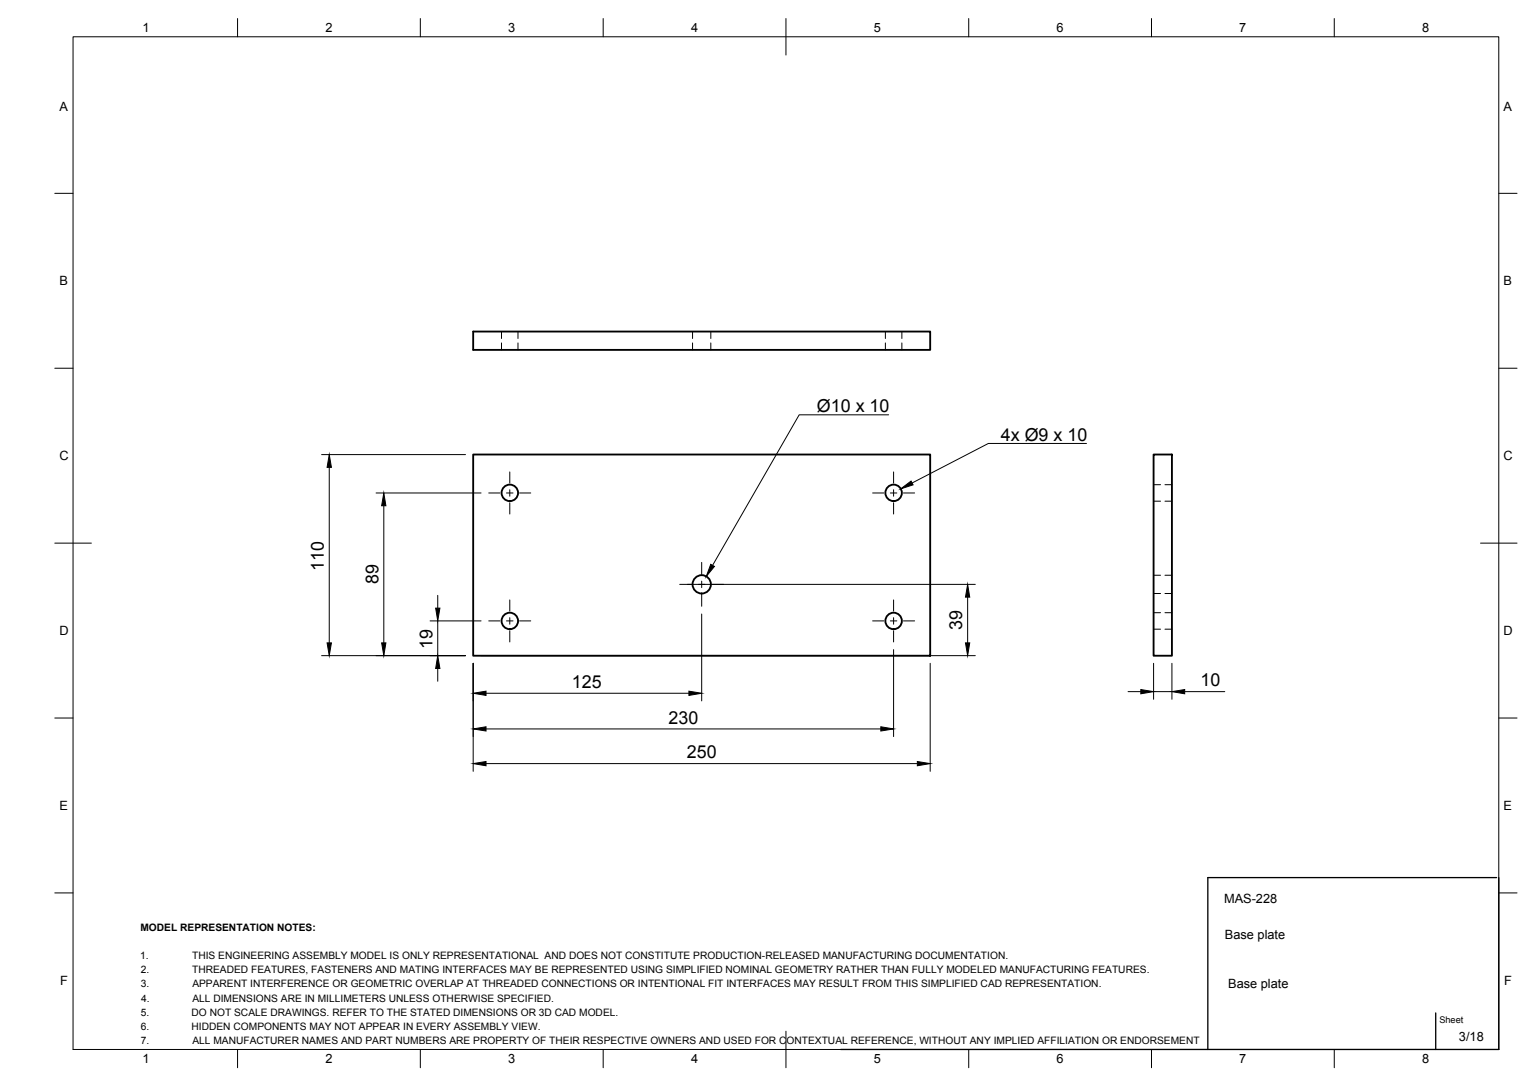
ISO-10303-21;
HEADER;
/* Generated by software containing ST-Developer
 * from STEP Tools, Inc. (www.steptools.com) 
 */

FILE_DESCRIPTION(
/* description */ ('Independent Peaucellier-Lipkin straight-line linkage. Radius arms 100
 mm, inversion-cell links 60 mm, crank radius and fixed-pivot spacing 
32 mm. Inversion constant 6400 mm squared, nominal output straight lin
e X=100 mm. Overhead bearing bridge clears the layered moving links. N
o accuracy or load rating assigned.'),
/* implementation_level */ '2;1');

FILE_NAME(
/* name */ 'Base plate.step',
/* time_stamp */ '2026-11-09T18:06:16-08:00',
/* author */ (''),
/* organization */ (''),
/* preprocessor_version */ 'ST-DEVELOPER v20.2',
/* originating_system */ 'Autodesk Translation Framework v15.17.0.0',
/* authorisation */ '');

FILE_SCHEMA (('AUTOMOTIVE_DESIGN { 1 0 10303 214 3 1 1 }'));
ENDSEC;

DATA;
#10=MECHANICAL_DESIGN_GEOMETRIC_PRESENTATION_REPRESENTATION('',(#282),#3581);
#248=SHAPE_REPRESENTATION_RELATIONSHIP('SRR','None',#3682,#265);
#265=ADVANCED_BREP_SHAPE_REPRESENTATION('',(#299),#3564);
#282=STYLED_ITEM('',(#3776),#299);
#299=MANIFOLD_SOLID_BREP('Body1',#1868);
#316=FACE_BOUND('',#546,.T.);
#317=FACE_BOUND('',#547,.T.);
#318=FACE_BOUND('',#548,.T.);
#319=FACE_BOUND('',#549,.T.);
#320=FACE_BOUND('',#550,.T.);
#321=FACE_BOUND('',#552,.T.);
#322=FACE_BOUND('',#553,.T.);
#323=FACE_BOUND('',#554,.T.);
#324=FACE_BOUND('',#555,.T.);
#325=FACE_BOUND('',#556,.T.);
#364=PLANE('',#2090);
#365=PLANE('',#2091);
#366=PLANE('',#2092);
#367=PLANE('',#2093);
#368=PLANE('',#2094);
#369=PLANE('',#2095);
#425=FACE_OUTER_BOUND('',#536,.T.);
#426=FACE_OUTER_BOUND('',#537,.T.);
#427=FACE_OUTER_BOUND('',#538,.T.);
#428=FACE_OUTER_BOUND('',#539,.T.);
#429=FACE_OUTER_BOUND('',#540,.T.);
#430=FACE_OUTER_BOUND('',#541,.T.);
#431=FACE_OUTER_BOUND('',#542,.T.);
#432=FACE_OUTER_BOUND('',#543,.T.);
#433=FACE_OUTER_BOUND('',#544,.T.);
#434=FACE_OUTER_BOUND('',#545,.T.);
#435=FACE_OUTER_BOUND('',#551,.T.);
#536=EDGE_LOOP('',(#1316,#1317,#1318,#1319));
#537=EDGE_LOOP('',(#1320,#1321,#1322,#1323));
#538=EDGE_LOOP('',(#1324,#1325,#1326,#1327));
#539=EDGE_LOOP('',(#1328,#1329,#1330,#1331));
#540=EDGE_LOOP('',(#1332,#1333,#1334,#1335));
#541=EDGE_LOOP('',(#1336,#1337,#1338,#1339));
#542=EDGE_LOOP('',(#1340,#1341,#1342,#1343));
#543=EDGE_LOOP('',(#1344,#1345,#1346,#1347));
#544=EDGE_LOOP('',(#1348,#1349,#1350,#1351));
#545=EDGE_LOOP('',(#1352,#1353,#1354,#1355));
#546=EDGE_LOOP('',(#1356));
#547=EDGE_LOOP('',(#1357));
#548=EDGE_LOOP('',(#1358));
#549=EDGE_LOOP('',(#1359));
#550=EDGE_LOOP('',(#1360));
#551=EDGE_LOOP('',(#1361,#1362,#1363,#1364));
#552=EDGE_LOOP('',(#1365));
#553=EDGE_LOOP('',(#1366));
#554=EDGE_LOOP('',(#1367));
#555=EDGE_LOOP('',(#1368));
#556=EDGE_LOOP('',(#1369));
#695=LINE('',#3035,#793);
#696=LINE('',#3041,#794);
#697=LINE('',#3047,#795);
#698=LINE('',#3053,#796);
#699=LINE('',#3059,#797);
#700=LINE('',#3064,#798);
#701=LINE('',#3066,#799);
#702=LINE('',#3068,#800);
#703=LINE('',#3069,#801);
#704=LINE('',#3072,#802);
#705=LINE('',#3074,#803);
#706=LINE('',#3075,#804);
#707=LINE('',#3078,#805);
#708=LINE('',#3080,#806);
#709=LINE('',#3081,#807);
#710=LINE('',#3083,#808);
#711=LINE('',#3084,#809);
#793=VECTOR('',#2367,4.5);
#794=VECTOR('',#2374,4.5);
#795=VECTOR('',#2381,4.5);
#796=VECTOR('',#2388,4.5);
#797=VECTOR('',#2395,5.);
#798=VECTOR('',#2400,10.);
#799=VECTOR('',#2401,10.);
#800=VECTOR('',#2402,10.);
#801=VECTOR('',#2403,10.);
#802=VECTOR('',#2406,10.);
#803=VECTOR('',#2407,10.);
#804=VECTOR('',#2408,10.);
#805=VECTOR('',#2411,10.);
#806=VECTOR('',#2412,10.);
#807=VECTOR('',#2413,10.);
#808=VECTOR('',#2416,10.);
#809=VECTOR('',#2417,10.);
#891=CIRCLE('',#2076,4.5);
#892=CIRCLE('',#2077,4.5);
#893=CIRCLE('',#2079,4.5);
#894=CIRCLE('',#2080,4.5);
#895=CIRCLE('',#2082,4.5);
#896=CIRCLE('',#2083,4.5);
#897=CIRCLE('',#2085,4.5);
#898=CIRCLE('',#2086,4.5);
#899=CIRCLE('',#2088,5.);
#900=CIRCLE('',#2089,5.);
#989=VERTEX_POINT('',#3032);
#990=VERTEX_POINT('',#3034);
#991=VERTEX_POINT('',#3038);
#992=VERTEX_POINT('',#3040);
#993=VERTEX_POINT('',#3044);
#994=VERTEX_POINT('',#3046);
#995=VERTEX_POINT('',#3050);
#996=VERTEX_POINT('',#3052);
#997=VERTEX_POINT('',#3056);
#998=VERTEX_POINT('',#3058);
#999=VERTEX_POINT('',#3062);
#1000=VERTEX_POINT('',#3063);
#1001=VERTEX_POINT('',#3065);
#1002=VERTEX_POINT('',#3067);
#1003=VERTEX_POINT('',#3071);
#1004=VERTEX_POINT('',#3073);
#1005=VERTEX_POINT('',#3077);
#1006=VERTEX_POINT('',#3079);
#1120=EDGE_CURVE('',#989,#989,#891,.T.);
#1121=EDGE_CURVE('',#989,#990,#695,.T.);
#1122=EDGE_CURVE('',#990,#990,#892,.T.);
#1123=EDGE_CURVE('',#991,#991,#893,.T.);
#1124=EDGE_CURVE('',#991,#992,#696,.T.);
#1125=EDGE_CURVE('',#992,#992,#894,.T.);
#1126=EDGE_CURVE('',#993,#993,#895,.T.);
#1127=EDGE_CURVE('',#993,#994,#697,.T.);
#1128=EDGE_CURVE('',#994,#994,#896,.T.);
#1129=EDGE_CURVE('',#995,#995,#897,.T.);
#1130=EDGE_CURVE('',#995,#996,#698,.T.);
#1131=EDGE_CURVE('',#996,#996,#898,.T.);
#1132=EDGE_CURVE('',#997,#997,#899,.T.);
#1133=EDGE_CURVE('',#997,#998,#699,.T.);
#1134=EDGE_CURVE('',#998,#998,#900,.T.);
#1135=EDGE_CURVE('',#999,#1000,#700,.F.);
#1136=EDGE_CURVE('',#1000,#1001,#701,.T.);
#1137=EDGE_CURVE('',#1002,#1001,#702,.F.);
#1138=EDGE_CURVE('',#999,#1002,#703,.F.);
#1139=EDGE_CURVE('',#1003,#999,#704,.F.);
#1140=EDGE_CURVE('',#1004,#1002,#705,.F.);
#1141=EDGE_CURVE('',#1003,#1004,#706,.F.);
#1142=EDGE_CURVE('',#1005,#1003,#707,.F.);
#1143=EDGE_CURVE('',#1006,#1004,#708,.F.);
#1144=EDGE_CURVE('',#1005,#1006,#709,.T.);
#1145=EDGE_CURVE('',#1000,#1005,#710,.F.);
#1146=EDGE_CURVE('',#1001,#1006,#711,.F.);
#1316=ORIENTED_EDGE('',*,*,#1120,.F.);
#1317=ORIENTED_EDGE('',*,*,#1121,.T.);
#1318=ORIENTED_EDGE('',*,*,#1122,.F.);
#1319=ORIENTED_EDGE('',*,*,#1121,.F.);
#1320=ORIENTED_EDGE('',*,*,#1123,.F.);
#1321=ORIENTED_EDGE('',*,*,#1124,.T.);
#1322=ORIENTED_EDGE('',*,*,#1125,.F.);
#1323=ORIENTED_EDGE('',*,*,#1124,.F.);
#1324=ORIENTED_EDGE('',*,*,#1126,.F.);
#1325=ORIENTED_EDGE('',*,*,#1127,.T.);
#1326=ORIENTED_EDGE('',*,*,#1128,.F.);
#1327=ORIENTED_EDGE('',*,*,#1127,.F.);
#1328=ORIENTED_EDGE('',*,*,#1129,.F.);
#1329=ORIENTED_EDGE('',*,*,#1130,.T.);
#1330=ORIENTED_EDGE('',*,*,#1131,.F.);
#1331=ORIENTED_EDGE('',*,*,#1130,.F.);
#1332=ORIENTED_EDGE('',*,*,#1132,.F.);
#1333=ORIENTED_EDGE('',*,*,#1133,.T.);
#1334=ORIENTED_EDGE('',*,*,#1134,.F.);
#1335=ORIENTED_EDGE('',*,*,#1133,.F.);
#1336=ORIENTED_EDGE('',*,*,#1135,.T.);
#1337=ORIENTED_EDGE('',*,*,#1136,.T.);
#1338=ORIENTED_EDGE('',*,*,#1137,.F.);
#1339=ORIENTED_EDGE('',*,*,#1138,.F.);
#1340=ORIENTED_EDGE('',*,*,#1139,.T.);
#1341=ORIENTED_EDGE('',*,*,#1138,.T.);
#1342=ORIENTED_EDGE('',*,*,#1140,.F.);
#1343=ORIENTED_EDGE('',*,*,#1141,.F.);
#1344=ORIENTED_EDGE('',*,*,#1142,.T.);
#1345=ORIENTED_EDGE('',*,*,#1141,.T.);
#1346=ORIENTED_EDGE('',*,*,#1143,.F.);
#1347=ORIENTED_EDGE('',*,*,#1144,.F.);
#1348=ORIENTED_EDGE('',*,*,#1145,.T.);
#1349=ORIENTED_EDGE('',*,*,#1144,.T.);
#1350=ORIENTED_EDGE('',*,*,#1146,.F.);
#1351=ORIENTED_EDGE('',*,*,#1136,.F.);
#1352=ORIENTED_EDGE('',*,*,#1146,.T.);
#1353=ORIENTED_EDGE('',*,*,#1143,.T.);
#1354=ORIENTED_EDGE('',*,*,#1140,.T.);
#1355=ORIENTED_EDGE('',*,*,#1137,.T.);
#1356=ORIENTED_EDGE('',*,*,#1132,.T.);
#1357=ORIENTED_EDGE('',*,*,#1129,.T.);
#1358=ORIENTED_EDGE('',*,*,#1126,.T.);
#1359=ORIENTED_EDGE('',*,*,#1123,.T.);
#1360=ORIENTED_EDGE('',*,*,#1120,.T.);
#1361=ORIENTED_EDGE('',*,*,#1145,.F.);
#1362=ORIENTED_EDGE('',*,*,#1135,.F.);
#1363=ORIENTED_EDGE('',*,*,#1139,.F.);
#1364=ORIENTED_EDGE('',*,*,#1142,.F.);
#1365=ORIENTED_EDGE('',*,*,#1134,.T.);
#1366=ORIENTED_EDGE('',*,*,#1131,.T.);
#1367=ORIENTED_EDGE('',*,*,#1128,.T.);
#1368=ORIENTED_EDGE('',*,*,#1125,.T.);
#1369=ORIENTED_EDGE('',*,*,#1122,.T.);
#1708=CYLINDRICAL_SURFACE('',#2075,4.5);
#1709=CYLINDRICAL_SURFACE('',#2078,4.5);
#1710=CYLINDRICAL_SURFACE('',#2081,4.5);
#1711=CYLINDRICAL_SURFACE('',#2084,4.5);
#1712=CYLINDRICAL_SURFACE('',#2087,5.);
#1757=ADVANCED_FACE('',(#425),#1708,.F.);
#1758=ADVANCED_FACE('',(#426),#1709,.F.);
#1759=ADVANCED_FACE('',(#427),#1710,.F.);
#1760=ADVANCED_FACE('',(#428),#1711,.F.);
#1761=ADVANCED_FACE('',(#429),#1712,.F.);
#1762=ADVANCED_FACE('',(#430),#364,.T.);
#1763=ADVANCED_FACE('',(#431),#365,.T.);
#1764=ADVANCED_FACE('',(#432),#366,.T.);
#1765=ADVANCED_FACE('',(#433),#367,.T.);
#1766=ADVANCED_FACE('',(#434,#316,#317,#318,#319,#320),#368,.T.);
#1767=ADVANCED_FACE('',(#435,#321,#322,#323,#324,#325),#369,.F.);
#1868=CLOSED_SHELL('',(#1757,#1758,#1759,#1760,#1761,#1762,#1763,#1764,
#1765,#1766,#1767));
#2074=AXIS2_PLACEMENT_3D('',#3030,#2361,#2362);
#2075=AXIS2_PLACEMENT_3D('',#3031,#2363,#2364);
#2076=AXIS2_PLACEMENT_3D('',#3033,#2365,#2366);
#2077=AXIS2_PLACEMENT_3D('',#3036,#2368,#2369);
#2078=AXIS2_PLACEMENT_3D('',#3037,#2370,#2371);
#2079=AXIS2_PLACEMENT_3D('',#3039,#2372,#2373);
#2080=AXIS2_PLACEMENT_3D('',#3042,#2375,#2376);
#2081=AXIS2_PLACEMENT_3D('',#3043,#2377,#2378);
#2082=AXIS2_PLACEMENT_3D('',#3045,#2379,#2380);
#2083=AXIS2_PLACEMENT_3D('',#3048,#2382,#2383);
#2084=AXIS2_PLACEMENT_3D('',#3049,#2384,#2385);
#2085=AXIS2_PLACEMENT_3D('',#3051,#2386,#2387);
#2086=AXIS2_PLACEMENT_3D('',#3054,#2389,#2390);
#2087=AXIS2_PLACEMENT_3D('',#3055,#2391,#2392);
#2088=AXIS2_PLACEMENT_3D('',#3057,#2393,#2394);
#2089=AXIS2_PLACEMENT_3D('',#3060,#2396,#2397);
#2090=AXIS2_PLACEMENT_3D('',#3061,#2398,#2399);
#2091=AXIS2_PLACEMENT_3D('',#3070,#2404,#2405);
#2092=AXIS2_PLACEMENT_3D('',#3076,#2409,#2410);
#2093=AXIS2_PLACEMENT_3D('',#3082,#2414,#2415);
#2094=AXIS2_PLACEMENT_3D('',#3085,#2418,#2419);
#2095=AXIS2_PLACEMENT_3D('',#3086,#2420,#2421);
#2361=DIRECTION('axis',(0.,0.,1.));
#2362=DIRECTION('refdir',(1.,0.,0.));
#2363=DIRECTION('center_axis',(0.,0.,-1.));
#2364=DIRECTION('ref_axis',(1.,0.,0.));
#2365=DIRECTION('center_axis',(0.,0.,-1.));
#2366=DIRECTION('ref_axis',(1.,0.,0.));
#2367=DIRECTION('',(0.,0.,-1.));
#2368=DIRECTION('center_axis',(0.,0.,1.));
#2369=DIRECTION('ref_axis',(1.,0.,0.));
#2370=DIRECTION('center_axis',(0.,0.,-1.));
#2371=DIRECTION('ref_axis',(1.,0.,0.));
#2372=DIRECTION('center_axis',(0.,0.,-1.));
#2373=DIRECTION('ref_axis',(1.,0.,0.));
#2374=DIRECTION('',(0.,0.,-1.));
#2375=DIRECTION('center_axis',(0.,0.,1.));
#2376=DIRECTION('ref_axis',(1.,0.,0.));
#2377=DIRECTION('center_axis',(0.,0.,-1.));
#2378=DIRECTION('ref_axis',(1.,0.,0.));
#2379=DIRECTION('center_axis',(0.,0.,-1.));
#2380=DIRECTION('ref_axis',(1.,0.,0.));
#2381=DIRECTION('',(0.,0.,-1.));
#2382=DIRECTION('center_axis',(0.,0.,1.));
#2383=DIRECTION('ref_axis',(1.,0.,0.));
#2384=DIRECTION('center_axis',(0.,0.,-1.));
#2385=DIRECTION('ref_axis',(1.,0.,0.));
#2386=DIRECTION('center_axis',(0.,0.,-1.));
#2387=DIRECTION('ref_axis',(1.,0.,0.));
#2388=DIRECTION('',(0.,0.,-1.));
#2389=DIRECTION('center_axis',(0.,0.,1.));
#2390=DIRECTION('ref_axis',(1.,0.,0.));
#2391=DIRECTION('center_axis',(0.,0.,-1.));
#2392=DIRECTION('ref_axis',(1.,0.,0.));
#2393=DIRECTION('center_axis',(0.,0.,-1.));
#2394=DIRECTION('ref_axis',(1.,0.,0.));
#2395=DIRECTION('',(0.,0.,-1.));
#2396=DIRECTION('center_axis',(0.,0.,1.));
#2397=DIRECTION('ref_axis',(1.,0.,0.));
#2398=DIRECTION('center_axis',(0.,1.,0.));
#2399=DIRECTION('ref_axis',(-1.,0.,0.));
#2400=DIRECTION('',(1.,0.,0.));
#2401=DIRECTION('',(0.,0.,1.));
#2402=DIRECTION('',(1.,0.,0.));
#2403=DIRECTION('',(0.,0.,-1.));
#2404=DIRECTION('center_axis',(1.,0.,0.));
#2405=DIRECTION('ref_axis',(0.,1.,0.));
#2406=DIRECTION('',(0.,-1.,0.));
#2407=DIRECTION('',(0.,-1.,0.));
#2408=DIRECTION('',(0.,0.,-1.));
#2409=DIRECTION('center_axis',(0.,-1.,0.));
#2410=DIRECTION('ref_axis',(1.,0.,0.));
#2411=DIRECTION('',(-1.,0.,0.));
#2412=DIRECTION('',(-1.,0.,0.));
#2413=DIRECTION('',(0.,0.,1.));
#2414=DIRECTION('center_axis',(-1.,0.,0.));
#2415=DIRECTION('ref_axis',(0.,-1.,0.));
#2416=DIRECTION('',(0.,1.,0.));
#2417=DIRECTION('',(0.,1.,0.));
#2418=DIRECTION('center_axis',(0.,0.,1.));
#2419=DIRECTION('ref_axis',(1.,0.,0.));
#2420=DIRECTION('center_axis',(0.,0.,1.));
#2421=DIRECTION('ref_axis',(1.,0.,0.));
#3030=CARTESIAN_POINT('',(0.,0.,0.));
#3031=CARTESIAN_POINT('Origin',(50.,-105.,5.));
#3032=CARTESIAN_POINT('',(45.5,-105.,10.));
#3033=CARTESIAN_POINT('Origin',(50.,-105.,10.));
#3034=CARTESIAN_POINT('',(45.5,-105.,0.));
#3035=CARTESIAN_POINT('',(45.5,-105.,5.));
#3036=CARTESIAN_POINT('Origin',(50.,-105.,0.));
#3037=CARTESIAN_POINT('Origin',(-20.,-105.,5.));
#3038=CARTESIAN_POINT('',(-24.5,-105.,10.));
#3039=CARTESIAN_POINT('Origin',(-20.,-105.,10.));
#3040=CARTESIAN_POINT('',(-24.5,-105.,0.));
#3041=CARTESIAN_POINT('',(-24.5,-105.,5.));
#3042=CARTESIAN_POINT('Origin',(-20.,-105.,0.));
#3043=CARTESIAN_POINT('Origin',(-20.,105.,5.));
#3044=CARTESIAN_POINT('',(-24.5,105.,10.));
#3045=CARTESIAN_POINT('Origin',(-20.,105.,10.));
#3046=CARTESIAN_POINT('',(-24.5,105.,0.));
#3047=CARTESIAN_POINT('',(-24.5,105.,5.));
#3048=CARTESIAN_POINT('Origin',(-20.,105.,0.));
#3049=CARTESIAN_POINT('Origin',(50.,105.,5.));
#3050=CARTESIAN_POINT('',(45.5,105.,10.));
#3051=CARTESIAN_POINT('Origin',(50.,105.,10.));
#3052=CARTESIAN_POINT('',(45.5,105.,0.));
#3053=CARTESIAN_POINT('',(45.5,105.,5.));
#3054=CARTESIAN_POINT('Origin',(50.,105.,0.));
#3055=CARTESIAN_POINT('Origin',(0.,0.,5.));
#3056=CARTESIAN_POINT('',(-5.,6.12323399573677E-16,10.));
#3057=CARTESIAN_POINT('Origin',(0.,0.,10.));
#3058=CARTESIAN_POINT('',(-5.,6.12323399573677E-16,0.));
#3059=CARTESIAN_POINT('',(-5.,6.12323399573677E-16,5.));
#3060=CARTESIAN_POINT('Origin',(0.,0.,0.));
#3061=CARTESIAN_POINT('Origin',(66.,125.,0.));
#3062=CARTESIAN_POINT('',(71.,125.,0.));
#3063=CARTESIAN_POINT('',(-39.,125.,0.));
#3064=CARTESIAN_POINT('',(41.,125.,0.));
#3065=CARTESIAN_POINT('',(-39.,125.,10.));
#3066=CARTESIAN_POINT('',(-39.,125.,0.));
#3067=CARTESIAN_POINT('',(71.,125.,10.));
#3068=CARTESIAN_POINT('',(41.,125.,10.));
#3069=CARTESIAN_POINT('',(71.,125.,0.));
#3070=CARTESIAN_POINT('Origin',(71.,-120.,0.));
#3071=CARTESIAN_POINT('',(71.,-125.,0.));
#3072=CARTESIAN_POINT('',(71.,-60.,0.));
#3073=CARTESIAN_POINT('',(71.,-125.,10.));
#3074=CARTESIAN_POINT('',(71.,-60.,10.));
#3075=CARTESIAN_POINT('',(71.,-125.,0.));
#3076=CARTESIAN_POINT('Origin',(-34.,-125.,0.));
#3077=CARTESIAN_POINT('',(-39.,-125.,0.));
#3078=CARTESIAN_POINT('',(-9.,-125.,0.));
#3079=CARTESIAN_POINT('',(-39.,-125.,10.));
#3080=CARTESIAN_POINT('',(-9.,-125.,10.));
#3081=CARTESIAN_POINT('',(-39.,-125.,0.));
#3082=CARTESIAN_POINT('Origin',(-39.,120.,0.));
#3083=CARTESIAN_POINT('',(-39.,60.,0.));
#3084=CARTESIAN_POINT('',(-39.,60.,10.));
#3085=CARTESIAN_POINT('Origin',(16.,0.,10.));
#3086=CARTESIAN_POINT('Origin',(16.,0.,0.));
#3545=UNCERTAINTY_MEASURE_WITH_UNIT(LENGTH_MEASURE(0.01),#3582,
'DISTANCE_ACCURACY_VALUE',
'Maximum model space distance between geometric entities at asserted c
onnectivities');
#3562=UNCERTAINTY_MEASURE_WITH_UNIT(LENGTH_MEASURE(0.01),#3582,
'DISTANCE_ACCURACY_VALUE',
'Maximum model space distance between geometric entities at asserted c
onnectivities');
#3564=(
GEOMETRIC_REPRESENTATION_CONTEXT(3)
GLOBAL_UNCERTAINTY_ASSIGNED_CONTEXT((#3545))
GLOBAL_UNIT_ASSIGNED_CONTEXT((#3582,#3584,#3585))
REPRESENTATION_CONTEXT('','3D')
);
#3581=(
GEOMETRIC_REPRESENTATION_CONTEXT(3)
GLOBAL_UNCERTAINTY_ASSIGNED_CONTEXT((#3562))
GLOBAL_UNIT_ASSIGNED_CONTEXT((#3582,#3584,#3585))
REPRESENTATION_CONTEXT('','3D')
);
#3582=(
LENGTH_UNIT()
NAMED_UNIT(*)
SI_UNIT(.MILLI.,.METRE.)
);
#3584=(
NAMED_UNIT(*)
PLANE_ANGLE_UNIT()
SI_UNIT($,.RADIAN.)
);
#3585=(
NAMED_UNIT(*)
SI_UNIT($,.STERADIAN.)
SOLID_ANGLE_UNIT()
);
#3587=SHAPE_DEFINITION_REPRESENTATION(#3605,#3682);
#3605=PRODUCT_DEFINITION_SHAPE('',$,#3701);
#3682=SHAPE_REPRESENTATION('',(#2074),#3564);
#3699=PRODUCT_DEFINITION_CONTEXT('part definition',#3755,'design');
#3701=PRODUCT_DEFINITION('Base plate','Base plate',#3719,#3699);
#3719=PRODUCT_DEFINITION_FORMATION('',$,#3758);
#3755=APPLICATION_CONTEXT(
'Core Data for Automotive Mechanical Design Process');
#3756=PRODUCT_CONTEXT('part definition',#3755,'mechanical');
#3758=PRODUCT('Base plate','Base plate','Base plate',(#3756));
#3776=PRESENTATION_STYLE_ASSIGNMENT((#3789));
#3789=SURFACE_STYLE_USAGE(.BOTH.,#3802);
#3802=SURFACE_SIDE_STYLE('',(#3815));
#3815=SURFACE_STYLE_FILL_AREA(#3828);
#3828=FILL_AREA_STYLE('Base gray',(#3841));
#3841=FILL_AREA_STYLE_COLOUR('Base gray',#3854);
#3854=COLOUR_RGB('Base gray',0.407843137254902,0.447058823529412,0.498039215686275);
ENDSEC;
END-ISO-10303-21;
